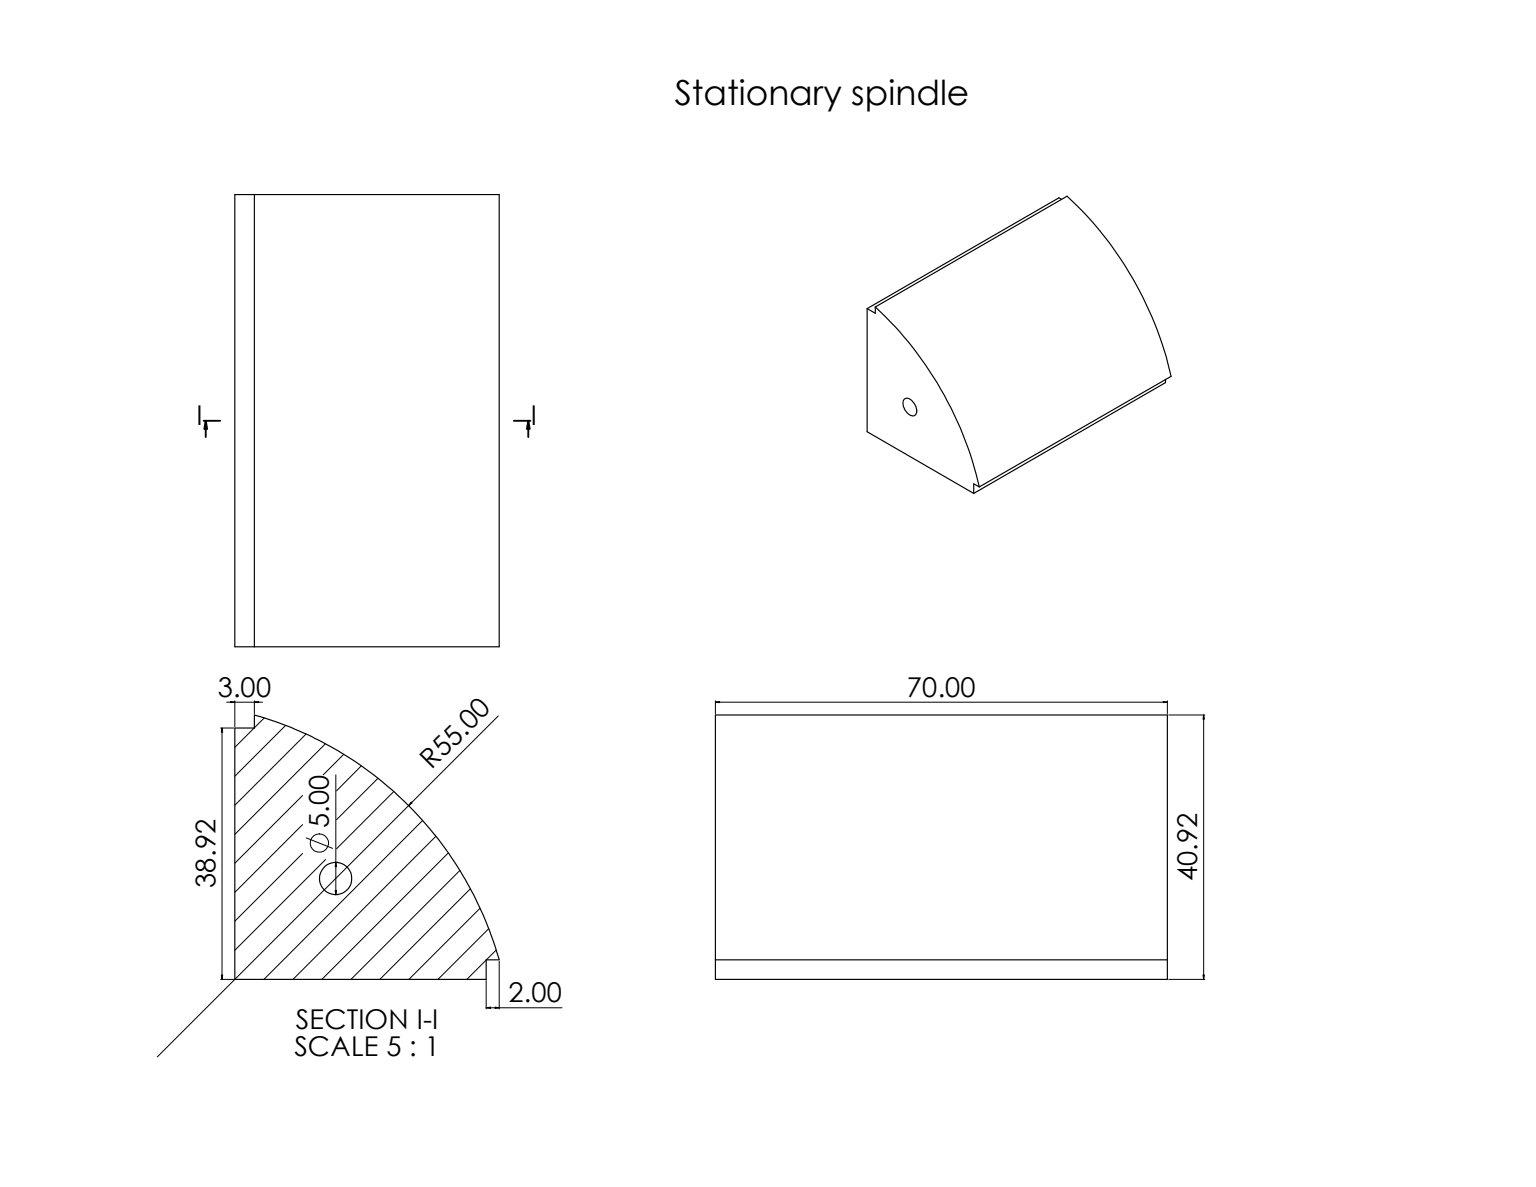
ISO-10303-21;
HEADER;
FILE_DESCRIPTION (('STEP AP214'),
    '1' );
FILE_NAME ('Stationary spindle.step',
    '2026-10-25T19:19:31',
    ( '' ),
    ( '' ),
    'SwSTEP 2.0',
    'SolidWorks 2025',
    '' );
FILE_SCHEMA (( 'AUTOMOTIVE_DESIGN' ));
ENDSEC;

DATA;
#4=DIRECTION ( 'NONE',  ( 1.000000000000000000, 1.776356839400250465E-15, 0.000000000000000000 ) ) ;
#22=CARTESIAN_POINT ( 'NONE',  ( 0.000000000000000000, 0.000000000000000000, -35.00000000000000000 ) ) ;
#73=AXIS2_PLACEMENT_3D ( 'NONE', #3304, #3763, #5645 ) ;
#75=MECHANICAL_DESIGN_GEOMETRIC_PRESENTATION_REPRESENTATION('',(#2849),#6131);
#80=DIRECTION ( 'NONE',  ( -0.000000000000000000, -0.000000000000000000, -1.000000000000000000 ) ) ;
#108=CARTESIAN_POINT ( 'NONE',  ( 12.00000000000000000, 12.00000000000000355, 35.00000000000000000 ) ) ;
#149=VERTEX_POINT ( 'NONE', #4105 ) ;
#164=EDGE_CURVE ( 'NONE', #4020, #3411, #5117, .T. ) ;
#178=SHAPE_DEFINITION_REPRESENTATION ( #473, #4081 ) ;
#253=EDGE_CURVE ( 'NONE', #2411, #1649, #3151, .T. ) ;
#263=ORIENTED_EDGE ( 'NONE', *, *, #5260, .F. ) ;
#271=ORIENTED_EDGE ( 'NONE', *, *, #5533, .F. ) ;
#308=DIRECTION ( 'NONE',  ( 1.000000000000000000, 0.000000000000000000, 0.000000000000000000 ) ) ;
#320=EDGE_CURVE ( 'NONE', #1017, #4020, #950, .T. ) ;
#327=DIRECTION ( 'NONE',  ( 0.000000000000000000, 0.000000000000000000, 1.000000000000000000 ) ) ;
#328=VERTEX_POINT ( 'NONE', #555 ) ;
#343=ORIENTED_EDGE ( 'NONE', *, *, #4753, .T. ) ;
#349=EDGE_LOOP ( 'NONE', ( #4550, #1268, #2494, #2612 ) ) ;
#376=CYLINDRICAL_SURFACE ( 'NONE', #2340, 2.499999999999998668 ) ;
#377=AXIS2_PLACEMENT_3D ( 'NONE', #1815, #1301, #327 ) ;
#383=FACE_OUTER_BOUND ( 'NONE', #5206, .T. ) ;
#397=( NAMED_UNIT ( * ) PLANE_ANGLE_UNIT ( ) SI_UNIT ( $, .RADIAN. ) );
#400=AXIS2_PLACEMENT_3D ( 'NONE', #1642, #1196, #3511 ) ;
#414=DIRECTION ( 'NONE',  ( 8.673617379883998001E-16, 1.000000000000000000, 0.000000000000000000 ) ) ;
#466=VECTOR ( 'NONE', #2853, 1000.000000000000000 ) ;
#468=ADVANCED_FACE ( 'NONE', ( #2082, #5872 ), #4008, .T. ) ;
#473=PRODUCT_DEFINITION_SHAPE ( 'NONE', 'NONE',  #5093 ) ;
#476=ADVANCED_FACE ( 'NONE', ( #3547 ), #1167, .F. ) ;
#509=CARTESIAN_POINT ( 'NONE',  ( 50.91502622129181788, 0.000000000000000000, 35.00000000000000000 ) ) ;
#520=ORIENTED_EDGE ( 'NONE', *, *, #3591, .F. ) ;
#527=CARTESIAN_POINT ( 'NONE',  ( 15.00000000000000000, 50.91502622129181788, -35.00000000000000000 ) ) ;
#544=CARTESIAN_POINT ( 'NONE',  ( 30.10043906316099083, 27.60043906316109386, -35.00000000000000000 ) ) ;
#550=( NAMED_UNIT ( * ) PLANE_ANGLE_UNIT ( ) SI_UNIT ( $, .RADIAN. ) );
#551=EDGE_LOOP ( 'NONE', ( #5803, #2026, #2863, #2751, #5984, #4013, #6009 ) ) ;
#555=CARTESIAN_POINT ( 'NONE',  ( 25.10043906316099083, 27.60043906316109386, 35.00000000000000000 ) ) ;
#568=CARTESIAN_POINT ( 'NONE',  ( -0.000000000000000000, 50.91502622129181788, -35.00000000000000000 ) ) ;
#650=ORIENTED_EDGE ( 'NONE', *, *, #4683, .F. ) ;
#667=ADVANCED_FACE ( 'NONE', ( #3633 ), #5550, .T. ) ;
#688=VERTEX_POINT ( 'NONE', #2707 ) ;
#706=CARTESIAN_POINT ( 'NONE',  ( 0.000000000000000000, 12.00000000000000355, 35.00000000000000000 ) ) ;
#720=VERTEX_POINT ( 'NONE', #3203 ) ;
#726=EDGE_LOOP ( 'NONE', ( #3570, #4220, #4699, #3819 ) ) ;
#751=EDGE_LOOP ( 'NONE', ( #4191, #5188, #5078, #271 ) ) ;
#755=CARTESIAN_POINT ( 'NONE',  ( 25.10043906316099083, 27.60043906316109386, -35.00000000000000000 ) ) ;
#781=DIRECTION ( 'NONE',  ( -0.000000000000000000, 0.000000000000000000, 1.000000000000000000 ) ) ;
#809=DIRECTION ( 'NONE',  ( -0.000000000000000000, -0.000000000000000000, -1.000000000000000000 ) ) ;
#829=PLANE ( 'NONE',  #4757 ) ;
#874=FACE_OUTER_BOUND ( 'NONE', #751, .T. ) ;
#896=CARTESIAN_POINT ( 'NONE',  ( 50.91502622129181788, 15.00000000000000355, 35.00000000000000000 ) ) ;
#922=DIRECTION ( 'NONE',  ( -1.000000000000000000, -8.673617379884027583E-15, 0.000000000000000000 ) ) ;
#923=( LENGTH_UNIT ( ) NAMED_UNIT ( * ) SI_UNIT ( .MILLI., .METRE. ) );
#950=LINE ( 'NONE', #2871, #1656 ) ;
#986=DIRECTION ( 'NONE',  ( 0.000000000000000000, 1.000000000000000000, -0.000000000000000000 ) ) ;
#995=AXIS2_PLACEMENT_3D ( 'NONE', #2420, #5267, #4 ) ;
#999=FACE_OUTER_BOUND ( 'NONE', #4574, .T. ) ;
#1017=VERTEX_POINT ( 'NONE', #4611 ) ;
#1024=LINE ( 'NONE', #5212, #2674 ) ;
#1036=EDGE_LOOP ( 'NONE', ( #3545, #2131, #2003, #343 ) ) ;
#1042=VERTEX_POINT ( 'NONE', #3696 ) ;
#1089=EDGE_CURVE ( 'NONE', #328, #5376, #1799, .T. ) ;
#1123=EDGE_CURVE ( 'NONE', #4796, #1042, #2187, .T. ) ;
#1143=ORIENTED_EDGE ( 'NONE', *, *, #1123, .T. ) ;
#1152=VECTOR ( 'NONE', #80, 1000.000000000000000 ) ;
#1167=CYLINDRICAL_SURFACE ( 'NONE', #400, 2.499999999999998668 ) ;
#1196=DIRECTION ( 'NONE',  ( -0.000000000000000000, -0.000000000000000000, -1.000000000000000000 ) ) ;
#1206=ORIENTED_EDGE ( 'NONE', *, *, #4650, .F. ) ;
#1222=EDGE_CURVE ( 'NONE', #3173, #149, #5703, .T. ) ;
#1229=LINE ( 'NONE', #4014, #5612 ) ;
#1243=ORIENTED_EDGE ( 'NONE', *, *, #5448, .T. ) ;
#1248=CARTESIAN_POINT ( 'NONE',  ( 52.91502622129182498, 15.00000000000001954, -35.00000000000000000 ) ) ;
#1262=ORIENTED_EDGE ( 'NONE', *, *, #5100, .T. ) ;
#1263=AXIS2_PLACEMENT_3D ( 'NONE', #509, #3316, #4204 ) ;
#1268=ORIENTED_EDGE ( 'NONE', *, *, #253, .T. ) ;
#1272=FACE_BOUND ( 'NONE', #4669, .T. ) ;
#1275=CARTESIAN_POINT ( 'NONE',  ( 0.000000000000000000, 50.91502622129181788, 35.00000000000000000 ) ) ;
#1278=PLANE ( 'NONE',  #1480 ) ;
#1295=ADVANCED_FACE ( 'NONE', ( #1993 ), #4736, .T. ) ;
#1301=DIRECTION ( 'NONE',  ( -1.000000000000000000, 0.000000000000000000, 0.000000000000000000 ) ) ;
#1345=VERTEX_POINT ( 'NONE', #5925 ) ;
#1354=CLOSED_SHELL ( 'NONE', ( #476, #1295, #3315, #667, #2484, #4606, #2119, #4414, #4024, #468, #2528 ) ) ;
#1413=EDGE_LOOP ( 'NONE', ( #5205, #2301, #5017, #1262 ) ) ;
#1452=VECTOR ( 'NONE', #414, 1000.000000000000000 ) ;
#1459=ORIENTED_EDGE ( 'NONE', *, *, #5260, .T. ) ;
#1480=AXIS2_PLACEMENT_3D ( 'NONE', #4135, #3179, #5087 ) ;
#1485=EDGE_CURVE ( 'NONE', #149, #5582, #5139, .T. ) ;
#1642=CARTESIAN_POINT ( 'NONE',  ( 27.60043906316099083, 27.60043906316109386, 35.00000000000000000 ) ) ;
#1649=VERTEX_POINT ( 'NONE', #544 ) ;
#1656=VECTOR ( 'NONE', #4326, 1000.000000000000000 ) ;
#1686=CARTESIAN_POINT ( 'NONE',  ( 15.00000000000000000, 50.91502622129181788, 35.00000000000000000 ) ) ;
#1706=LINE ( 'NONE', #5609, #2127 ) ;
#1747=( GEOMETRIC_REPRESENTATION_CONTEXT ( 3 ) GLOBAL_UNCERTAINTY_ASSIGNED_CONTEXT ( ( #1880 ) ) GLOBAL_UNIT_ASSIGNED_CONTEXT ( ( #923, #397, #5586 ) ) REPRESENTATION_CONTEXT ( 'NONE', 'WORKASPACE' ) );
#1781=ORIENTED_EDGE ( 'NONE', *, *, #2108, .T. ) ;
#1799=LINE ( 'NONE', #2212, #4144 ) ;
#1800=LINE ( 'NONE', #896, #1152 ) ;
#1815=CARTESIAN_POINT ( 'NONE',  ( 12.00000000000000000, 0.000000000000000000, 35.00000000000000000 ) ) ;
#1844=CARTESIAN_POINT ( 'NONE',  ( 50.91502622129181788, 0.000000000000000000, -35.00000000000000000 ) ) ;
#1847=EDGE_CURVE ( 'NONE', #720, #3173, #3504, .T. ) ;
#1862=VECTOR ( 'NONE', #5992, 1000.000000000000000 ) ;
#1871=AXIS2_PLACEMENT_3D ( 'NONE', #22, #4840, #2930 ) ;
#1880=UNCERTAINTY_MEASURE_WITH_UNIT (LENGTH_MEASURE( 1.000000000000000082E-05 ), #923, 'distance_accuracy_value', 'NONE');
#1908=CARTESIAN_POINT ( 'NONE',  ( 12.00000000000000000, 0.000000000000000000, -35.00000000000000000 ) ) ;
#1944=CARTESIAN_POINT ( 'NONE',  ( 12.00000000000000000, 50.91502622129181788, -35.00000000000000000 ) ) ;
#1946=PRODUCT_DEFINITION_CONTEXT ( 'detailed design', #2778, 'design' ) ;
#1993=FACE_OUTER_BOUND ( 'NONE', #5463, .T. ) ;
#2003=ORIENTED_EDGE ( 'NONE', *, *, #5024, .T. ) ;
#2026=ORIENTED_EDGE ( 'NONE', *, *, #1123, .F. ) ;
#2082=FACE_BOUND ( 'NONE', #2328, .T. ) ;
#2108=EDGE_CURVE ( 'NONE', #1042, #4214, #5689, .T. ) ;
#2119=ADVANCED_FACE ( 'NONE', ( #4686 ), #4342, .T. ) ;
#2126=EDGE_CURVE ( 'NONE', #3411, #4200, #3871, .T. ) ;
#2127=VECTOR ( 'NONE', #2742, 1000.000000000000000 ) ;
#2131=ORIENTED_EDGE ( 'NONE', *, *, #5100, .F. ) ;
#2133=AXIS2_PLACEMENT_3D ( 'NONE', #3258, #4207, #3289 ) ;
#2139=CIRCLE ( 'NONE', #2944, 2.499999999999998668 ) ;
#2153=MANIFOLD_SOLID_BREP ( 'Boss-Extrude5', #1354 ) ;
#2187=LINE ( 'NONE', #4076, #1862 ) ;
#2212=CARTESIAN_POINT ( 'NONE',  ( 25.10043906316099083, 27.60043906316109386, 35.00000000000000000 ) ) ;
#2259=VECTOR ( 'NONE', #5084, 1000.000000000000000 ) ;
#2263=VECTOR ( 'NONE', #5671, 1000.000000000000000 ) ;
#2276=SHAPE_REPRESENTATION_RELATIONSHIP ( 'NONE' , 'NONE' ,  #4081, #3579 ) ;
#2291=CARTESIAN_POINT ( 'NONE',  ( 30.10043906316099083, 27.60043906316109386, 35.00000000000000000 ) ) ;
#2301=ORIENTED_EDGE ( 'NONE', *, *, #320, .F. ) ;
#2316=DIRECTION ( 'NONE',  ( 0.000000000000000000, -1.000000000000000000, 0.000000000000000000 ) ) ;
#2328=EDGE_LOOP ( 'NONE', ( #1206, #650 ) ) ;
#2330=DIRECTION ( 'NONE',  ( 1.000000000000000000, 0.000000000000000000, 0.000000000000000000 ) ) ;
#2331=VECTOR ( 'NONE', #4361, 1000.000000000000000 ) ;
#2336=LINE ( 'NONE', #2470, #2331 ) ;
#2340=AXIS2_PLACEMENT_3D ( 'NONE', #5539, #2755, #3617 ) ;
#2387=DIRECTION ( 'NONE',  ( 0.000000000000000000, -0.000000000000000000, -1.000000000000000000 ) ) ;
#2397=EDGE_CURVE ( 'NONE', #5277, #4214, #3713, .T. ) ;
#2411=VERTEX_POINT ( 'NONE', #2291 ) ;
#2416=PLANE ( 'NONE',  #2723 ) ;
#2420=CARTESIAN_POINT ( 'NONE',  ( 0.000000000000000000, 0.000000000000000000, 35.00000000000000000 ) ) ;
#2470=CARTESIAN_POINT ( 'NONE',  ( 0.000000000000000000, 12.00000000000000355, -35.00000000000000000 ) ) ;
#2484=ADVANCED_FACE ( 'NONE', ( #5600 ), #5630, .T. ) ;
#2494=ORIENTED_EDGE ( 'NONE', *, *, #2773, .F. ) ;
#2514=DIRECTION ( 'NONE',  ( 1.000000000000000000, 0.000000000000000000, 0.000000000000000000 ) ) ;
#2528=ADVANCED_FACE ( 'NONE', ( #1272, #383 ), #829, .F. ) ;
#2553=CIRCLE ( 'NONE', #4959, 2.499999999999998668 ) ;
#2567=EDGE_CURVE ( 'NONE', #1042, #1017, #2577, .T. ) ;
#2577=CIRCLE ( 'NONE', #995, 55.00000000000002132 ) ;
#2599=EDGE_LOOP ( 'NONE', ( #4253, #2986, #1143, #1781 ) ) ;
#2612=ORIENTED_EDGE ( 'NONE', *, *, #1089, .F. ) ;
#2620=DIRECTION ( 'NONE',  ( -0.000000000000000000, 0.000000000000000000, 1.000000000000000000 ) ) ;
#2633=ORIENTED_EDGE ( 'NONE', *, *, #1485, .T. ) ;
#2674=VECTOR ( 'NONE', #5648, 1000.000000000000000 ) ;
#2704=DIRECTION ( 'NONE',  ( 1.000000000000000000, 0.000000000000000000, 0.000000000000000000 ) ) ;
#2707=CARTESIAN_POINT ( 'NONE',  ( 50.91502622129181788, 15.00000000000000355, 35.00000000000000000 ) ) ;
#2723=AXIS2_PLACEMENT_3D ( 'NONE', #4305, #5289, #2387 ) ;
#2735=FACE_OUTER_BOUND ( 'NONE', #1413, .T. ) ;
#2738=VECTOR ( 'NONE', #4018, 1000.000000000000000 ) ;
#2742=DIRECTION ( 'NONE',  ( 0.000000000000000000, -1.000000000000000000, 0.000000000000000000 ) ) ;
#2751=ORIENTED_EDGE ( 'NONE', *, *, #1222, .F. ) ;
#2755=DIRECTION ( 'NONE',  ( -0.000000000000000000, -0.000000000000000000, -1.000000000000000000 ) ) ;
#2773=EDGE_CURVE ( 'NONE', #5376, #1649, #2553, .T. ) ;
#2778=APPLICATION_CONTEXT ( 'automotive_design' ) ;
#2783=ORIENTED_EDGE ( 'NONE', *, *, #2397, .T. ) ;
#2816=CARTESIAN_POINT ( 'NONE',  ( 15.00000000000000178, 52.91502622129183209, 35.00000000000000000 ) ) ;
#2845=PRODUCT ( 'Stationary spindle', 'Stationary spindle', '', ( #3575 ) ) ;
#2849=STYLED_ITEM('',(#6170),#2153);
#2853=DIRECTION ( 'NONE',  ( 0.000000000000000000, 1.000000000000000000, -0.000000000000000000 ) ) ;
#2863=ORIENTED_EDGE ( 'NONE', *, *, #4845, .F. ) ;
#2871=CARTESIAN_POINT ( 'NONE',  ( 52.91502622129182498, 15.00000000000001954, 35.00000000000000000 ) ) ;
#2896=ORIENTED_EDGE ( 'NONE', *, *, #5448, .F. ) ;
#2910=CARTESIAN_POINT ( 'NONE',  ( 27.60043906316099083, 27.60043906316109386, 35.00000000000000000 ) ) ;
#2930=DIRECTION ( 'NONE',  ( 1.000000000000000000, 1.776356839400250465E-15, 0.000000000000000000 ) ) ;
#2944=AXIS2_PLACEMENT_3D ( 'NONE', #5384, #781, #3932 ) ;
#2986=ORIENTED_EDGE ( 'NONE', *, *, #5982, .F. ) ;
#3053=DIRECTION ( 'NONE',  ( 1.000000000000000000, 0.000000000000000000, 0.000000000000000000 ) ) ;
#3056=VECTOR ( 'NONE', #922, 1000.000000000000000 ) ;
#3151=LINE ( 'NONE', #5778, #4153 ) ;
#3168=ORIENTED_EDGE ( 'NONE', *, *, #2108, .F. ) ;
#3173=VERTEX_POINT ( 'NONE', #4459 ) ;
#3174=DIRECTION ( 'NONE',  ( -0.000000000000000000, 0.000000000000000000, 1.000000000000000000 ) ) ;
#3179=DIRECTION ( 'NONE',  ( -1.000000000000000000, 8.673617379883998001E-16, 0.000000000000000000 ) ) ;
#3203=CARTESIAN_POINT ( 'NONE',  ( 50.91502622129181788, 12.00000000000000355, 35.00000000000000000 ) ) ;
#3228=CARTESIAN_POINT ( 'NONE',  ( 0.000000000000000000, 0.000000000000000000, -35.00000000000000000 ) ) ;
#3258=CARTESIAN_POINT ( 'NONE',  ( 27.60043906316099083, 27.60043906316109386, -35.00000000000000000 ) ) ;
#3260=AXIS2_PLACEMENT_3D ( 'NONE', #5642, #3274, #5179 ) ;
#3263=CARTESIAN_POINT ( 'NONE',  ( 14.99999999999995559, -1.301042606982595854E-14, -35.00000000000000000 ) ) ;
#3274=DIRECTION ( 'NONE',  ( -0.000000000000000000, -0.000000000000000000, -1.000000000000000000 ) ) ;
#3289=DIRECTION ( 'NONE',  ( 1.000000000000000000, 0.000000000000000000, 0.000000000000000000 ) ) ;
#3302=CARTESIAN_POINT ( 'NONE',  ( 12.00000000000000000, 0.000000000000000000, 35.00000000000000000 ) ) ;
#3304=CARTESIAN_POINT ( 'NONE',  ( 0.000000000000000000, 0.000000000000000000, 0.000000000000000000 ) ) ;
#3315=ADVANCED_FACE ( 'NONE', ( #5497 ), #1278, .T. ) ;
#3316=DIRECTION ( 'NONE',  ( 1.000000000000000000, 0.000000000000000000, -0.000000000000000000 ) ) ;
#3320=ORIENTED_EDGE ( 'NONE', *, *, #4753, .F. ) ;
#3350=EDGE_CURVE ( 'NONE', #3173, #1345, #4731, .T. ) ;
#3402=CARTESIAN_POINT ( 'NONE',  ( 15.00000000000000000, 50.91502622129181788, 35.00000000000000000 ) ) ;
#3411=VERTEX_POINT ( 'NONE', #5638 ) ;
#3504=LINE ( 'NONE', #706, #3723 ) ;
#3511=DIRECTION ( 'NONE',  ( -1.000000000000000000, 0.000000000000000000, 0.000000000000000000 ) ) ;
#3516=CIRCLE ( 'NONE', #5025, 2.499999999999998668 ) ;
#3532=VECTOR ( 'NONE', #5287, 1000.000000000000000 ) ;
#3536=PRODUCT_DEFINITION_FORMATION_WITH_SPECIFIED_SOURCE ( 'ANY', '', #2845, .NOT_KNOWN. ) ;
#3545=ORIENTED_EDGE ( 'NONE', *, *, #2126, .F. ) ;
#3547=FACE_OUTER_BOUND ( 'NONE', #349, .T. ) ;
#3570=ORIENTED_EDGE ( 'NONE', *, *, #4538, .F. ) ;
#3573=CARTESIAN_POINT ( 'NONE',  ( 12.00000000000000000, 50.91502622129181788, 35.00000000000000000 ) ) ;
#3575=PRODUCT_CONTEXT ( 'NONE', #5891, 'mechanical' ) ;
#3579=ADVANCED_BREP_SHAPE_REPRESENTATION ( '', ( #2153, #73 ), #1747 ) ;
#3591=EDGE_CURVE ( 'NONE', #4214, #4020, #5569, .T. ) ;
#3617=DIRECTION ( 'NONE',  ( -1.000000000000000000, 0.000000000000000000, 0.000000000000000000 ) ) ;
#3633=FACE_OUTER_BOUND ( 'NONE', #726, .T. ) ;
#3653=EDGE_CURVE ( 'NONE', #1017, #688, #1024, .T. ) ;
#3696=CARTESIAN_POINT ( 'NONE',  ( 15.00000000000000178, 52.91502622129183209, 35.00000000000000000 ) ) ;
#3713=LINE ( 'NONE', #3263, #1452 ) ;
#3722=CARTESIAN_POINT ( 'NONE',  ( 27.60043906316099083, 27.60043906316109386, -35.00000000000000000 ) ) ;
#3723=VECTOR ( 'NONE', #4476, 1000.000000000000000 ) ;
#3739=AXIS2_PLACEMENT_3D ( 'NONE', #3918, #2620, #3053 ) ;
#3763=DIRECTION ( 'NONE',  ( 0.000000000000000000, 0.000000000000000000, 1.000000000000000000 ) ) ;
#3771=ORIENTED_EDGE ( 'NONE', *, *, #4538, .T. ) ;
#3817=CIRCLE ( 'NONE', #2133, 2.499999999999998668 ) ;
#3819=ORIENTED_EDGE ( 'NONE', *, *, #5982, .T. ) ;
#3845=EDGE_LOOP ( 'NONE', ( #2896, #5965, #5999, #2633 ) ) ;
#3871=LINE ( 'NONE', #1844, #4743 ) ;
#3889=DIRECTION ( 'NONE',  ( -0.000000000000000000, -0.000000000000000000, -1.000000000000000000 ) ) ;
#3918=CARTESIAN_POINT ( 'NONE',  ( 0.000000000000000000, 0.000000000000000000, 35.00000000000000000 ) ) ;
#3932=DIRECTION ( 'NONE',  ( 1.000000000000000000, 0.000000000000000000, 0.000000000000000000 ) ) ;
#4008=PLANE ( 'NONE',  #3739 ) ;
#4013=ORIENTED_EDGE ( 'NONE', *, *, #5024, .F. ) ;
#4014=CARTESIAN_POINT ( 'NONE',  ( 0.000000000000000000, 50.91502622129181788, 35.00000000000000000 ) ) ;
#4018=DIRECTION ( 'NONE',  ( -0.000000000000000000, -0.000000000000000000, -1.000000000000000000 ) ) ;
#4020=VERTEX_POINT ( 'NONE', #1248 ) ;
#4024=ADVANCED_FACE ( 'NONE', ( #2735 ), #5143, .T. ) ;
#4030=ORIENTED_EDGE ( 'NONE', *, *, #2773, .T. ) ;
#4076=CARTESIAN_POINT ( 'NONE',  ( 14.99999999999995559, -1.301042606982595854E-14, 35.00000000000000000 ) ) ;
#4081=SHAPE_REPRESENTATION ( 'Stationary spindle', ( #73 ), #1747 ) ;
#4105=CARTESIAN_POINT ( 'NONE',  ( 12.00000000000000000, 50.91502622129181788, 35.00000000000000000 ) ) ;
#4135=CARTESIAN_POINT ( 'NONE',  ( 14.99999999999995559, -1.301042606982595854E-14, 35.00000000000000000 ) ) ;
#4144=VECTOR ( 'NONE', #809, 1000.000000000000000 ) ;
#4153=VECTOR ( 'NONE', #3889, 1000.000000000000000 ) ;
#4191=ORIENTED_EDGE ( 'NONE', *, *, #253, .F. ) ;
#4200=VERTEX_POINT ( 'NONE', #5365 ) ;
#4202=ORIENTED_EDGE ( 'NONE', *, *, #1847, .T. ) ;
#4204=DIRECTION ( 'NONE',  ( -0.000000000000000000, 0.000000000000000000, -1.000000000000000000 ) ) ;
#4207=DIRECTION ( 'NONE',  ( -0.000000000000000000, 0.000000000000000000, 1.000000000000000000 ) ) ;
#4214=VERTEX_POINT ( 'NONE', #5797 ) ;
#4220=ORIENTED_EDGE ( 'NONE', *, *, #1485, .F. ) ;
#4231=VECTOR ( 'NONE', #4786, 1000.000000000000000 ) ;
#4253=ORIENTED_EDGE ( 'NONE', *, *, #2397, .F. ) ;
#4305=CARTESIAN_POINT ( 'NONE',  ( 0.000000000000000000, 12.00000000000000355, 35.00000000000000000 ) ) ;
#4326=DIRECTION ( 'NONE',  ( -0.000000000000000000, -0.000000000000000000, -1.000000000000000000 ) ) ;
#4342=PLANE ( 'NONE',  #1263 ) ;
#4361=DIRECTION ( 'NONE',  ( -1.000000000000000000, 0.000000000000000000, 0.000000000000000000 ) ) ;
#4374=LINE ( 'NONE', #568, #5432 ) ;
#4414=ADVANCED_FACE ( 'NONE', ( #874 ), #376, .F. ) ;
#4459=CARTESIAN_POINT ( 'NONE',  ( 12.00000000000000000, 12.00000000000000355, 35.00000000000000000 ) ) ;
#4476=DIRECTION ( 'NONE',  ( -1.000000000000000000, 0.000000000000000000, 0.000000000000000000 ) ) ;
#4538=EDGE_CURVE ( 'NONE', #5582, #5277, #4374, .T. ) ;
#4540=ORIENTED_EDGE ( 'NONE', *, *, #164, .T. ) ;
#4550=ORIENTED_EDGE ( 'NONE', *, *, #4650, .T. ) ;
#4574=EDGE_LOOP ( 'NONE', ( #263, #3320, #4202, #5299 ) ) ;
#4604=DIRECTION ( 'NONE',  ( 0.000000000000000000, 1.000000000000000000, 0.000000000000000000 ) ) ;
#4606=ADVANCED_FACE ( 'NONE', ( #999 ), #2416, .T. ) ;
#4611=CARTESIAN_POINT ( 'NONE',  ( 52.91502622129182498, 15.00000000000001954, 35.00000000000000000 ) ) ;
#4638=DIRECTION ( 'NONE',  ( 1.000000000000000000, 8.673617379884027583E-15, 0.000000000000000000 ) ) ;
#4647=AXIS2_PLACEMENT_3D ( 'NONE', #1275, #4604, #5141 ) ;
#4650=EDGE_CURVE ( 'NONE', #328, #2411, #3516, .T. ) ;
#4669=EDGE_LOOP ( 'NONE', ( #4030, #4888 ) ) ;
#4683=EDGE_CURVE ( 'NONE', #2411, #328, #2139, .T. ) ;
#4686=FACE_OUTER_BOUND ( 'NONE', #1036, .T. ) ;
#4688=UNCERTAINTY_MEASURE_WITH_UNIT (LENGTH_MEASURE( 1.000000000000000082E-05 ), #5652, 'distance_accuracy_value', 'NONE');
#4699=ORIENTED_EDGE ( 'NONE', *, *, #4845, .T. ) ;
#4731=LINE ( 'NONE', #108, #2263 ) ;
#4736=CYLINDRICAL_SURFACE ( 'NONE', #3260, 55.00000000000002132 ) ;
#4743=VECTOR ( 'NONE', #2316, 1000.000000000000000 ) ;
#4753=EDGE_CURVE ( 'NONE', #720, #4200, #5410, .T. ) ;
#4757=AXIS2_PLACEMENT_3D ( 'NONE', #3228, #3174, #2704 ) ;
#4786=DIRECTION ( 'NONE',  ( -0.000000000000000000, -0.000000000000000000, -1.000000000000000000 ) ) ;
#4796=VERTEX_POINT ( 'NONE', #1686 ) ;
#4840=DIRECTION ( 'NONE',  ( 0.000000000000000000, -0.000000000000000000, -1.000000000000000000 ) ) ;
#4845=EDGE_CURVE ( 'NONE', #149, #4796, #1229, .T. ) ;
#4888=ORIENTED_EDGE ( 'NONE', *, *, #5533, .T. ) ;
#4959=AXIS2_PLACEMENT_3D ( 'NONE', #3722, #6105, #2330 ) ;
#5017=ORIENTED_EDGE ( 'NONE', *, *, #3653, .T. ) ;
#5024=EDGE_CURVE ( 'NONE', #688, #720, #1706, .T. ) ;
#5025=AXIS2_PLACEMENT_3D ( 'NONE', #2910, #5787, #5882 ) ;
#5032=AXIS2_PLACEMENT_3D ( 'NONE', #5496, #5110, #4638 ) ;
#5048=ORIENTED_EDGE ( 'NONE', *, *, #2126, .T. ) ;
#5058=ORIENTED_EDGE ( 'NONE', *, *, #2567, .T. ) ;
#5078=ORIENTED_EDGE ( 'NONE', *, *, #1089, .T. ) ;
#5084=DIRECTION ( 'NONE',  ( -0.000000000000000000, -0.000000000000000000, -1.000000000000000000 ) ) ;
#5087=DIRECTION ( 'NONE',  ( -8.673617379883998001E-16, -1.000000000000000000, 0.000000000000000000 ) ) ;
#5093=PRODUCT_DEFINITION ( 'UNKNOWN', '', #3536, #1946 ) ;
#5100=EDGE_CURVE ( 'NONE', #688, #3411, #1800, .T. ) ;
#5110=DIRECTION ( 'NONE',  ( 8.673617379884027583E-15, -1.000000000000000000, 0.000000000000000000 ) ) ;
#5117=LINE ( 'NONE', #6081, #3056 ) ;
#5139=LINE ( 'NONE', #3573, #2259 ) ;
#5141=DIRECTION ( 'NONE',  ( 0.000000000000000000, -0.000000000000000000, 1.000000000000000000 ) ) ;
#5143=PLANE ( 'NONE',  #5032 ) ;
#5179=DIRECTION ( 'NONE',  ( -1.000000000000000000, 0.000000000000000000, 0.000000000000000000 ) ) ;
#5188=ORIENTED_EDGE ( 'NONE', *, *, #4683, .T. ) ;
#5205=ORIENTED_EDGE ( 'NONE', *, *, #164, .F. ) ;
#5206=EDGE_LOOP ( 'NONE', ( #5543, #4540, #5048, #1459, #1243, #3771, #2783 ) ) ;
#5212=CARTESIAN_POINT ( 'NONE',  ( -1.301042606982566193E-13, 14.99999999999956124, 35.00000000000000000 ) ) ;
#5260=EDGE_CURVE ( 'NONE', #4200, #1345, #2336, .T. ) ;
#5267=DIRECTION ( 'NONE',  ( 0.000000000000000000, -0.000000000000000000, -1.000000000000000000 ) ) ;
#5277=VERTEX_POINT ( 'NONE', #527 ) ;
#5287=DIRECTION ( 'NONE',  ( -0.000000000000000000, -0.000000000000000000, -1.000000000000000000 ) ) ;
#5289=DIRECTION ( 'NONE',  ( 0.000000000000000000, -1.000000000000000000, 0.000000000000000000 ) ) ;
#5299=ORIENTED_EDGE ( 'NONE', *, *, #3350, .T. ) ;
#5304=ORIENTED_EDGE ( 'NONE', *, *, #320, .T. ) ;
#5365=CARTESIAN_POINT ( 'NONE',  ( 50.91502622129181788, 12.00000000000000355, -35.00000000000000000 ) ) ;
#5376=VERTEX_POINT ( 'NONE', #755 ) ;
#5384=CARTESIAN_POINT ( 'NONE',  ( 27.60043906316099083, 27.60043906316109386, 35.00000000000000000 ) ) ;
#5410=LINE ( 'NONE', #5477, #2738 ) ;
#5432=VECTOR ( 'NONE', #2514, 1000.000000000000000 ) ;
#5448=EDGE_CURVE ( 'NONE', #1345, #5582, #6092, .T. ) ;
#5463=EDGE_LOOP ( 'NONE', ( #520, #3168, #5058, #5304 ) ) ;
#5477=CARTESIAN_POINT ( 'NONE',  ( 50.91502622129181788, 12.00000000000000355, 35.00000000000000000 ) ) ;
#5496=CARTESIAN_POINT ( 'NONE',  ( -1.301042606982566193E-13, 14.99999999999956124, 35.00000000000000000 ) ) ;
#5497=FACE_OUTER_BOUND ( 'NONE', #2599, .T. ) ;
#5533=EDGE_CURVE ( 'NONE', #1649, #5376, #3817, .T. ) ;
#5539=CARTESIAN_POINT ( 'NONE',  ( 27.60043906316099083, 27.60043906316109386, 35.00000000000000000 ) ) ;
#5543=ORIENTED_EDGE ( 'NONE', *, *, #3591, .T. ) ;
#5550=PLANE ( 'NONE',  #4647 ) ;
#5569=CIRCLE ( 'NONE', #1871, 55.00000000000002132 ) ;
#5582=VERTEX_POINT ( 'NONE', #1944 ) ;
#5586=( NAMED_UNIT ( * ) SI_UNIT ( $, .STERADIAN. ) SOLID_ANGLE_UNIT ( ) );
#5600=FACE_OUTER_BOUND ( 'NONE', #3845, .T. ) ;
#5609=CARTESIAN_POINT ( 'NONE',  ( 50.91502622129181788, 0.000000000000000000, 35.00000000000000000 ) ) ;
#5612=VECTOR ( 'NONE', #308, 1000.000000000000000 ) ;
#5630=PLANE ( 'NONE',  #377 ) ;
#5638=CARTESIAN_POINT ( 'NONE',  ( 50.91502622129181788, 15.00000000000000355, -35.00000000000000000 ) ) ;
#5642=CARTESIAN_POINT ( 'NONE',  ( 0.000000000000000000, 0.000000000000000000, 35.00000000000000000 ) ) ;
#5645=DIRECTION ( 'NONE',  ( 1.000000000000000000, 0.000000000000000000, 0.000000000000000000 ) ) ;
#5648=DIRECTION ( 'NONE',  ( -1.000000000000000000, -8.673617379884027583E-15, 0.000000000000000000 ) ) ;
#5652=( LENGTH_UNIT ( ) NAMED_UNIT ( * ) SI_UNIT ( .MILLI., .METRE. ) );
#5657=VECTOR ( 'NONE', #986, 1000.000000000000000 ) ;
#5671=DIRECTION ( 'NONE',  ( -0.000000000000000000, -0.000000000000000000, -1.000000000000000000 ) ) ;
#5689=LINE ( 'NONE', #2816, #4231 ) ;
#5703=LINE ( 'NONE', #3302, #5657 ) ;
#5750=LINE ( 'NONE', #3402, #3532 ) ;
#5778=CARTESIAN_POINT ( 'NONE',  ( 30.10043906316099083, 27.60043906316109386, 35.00000000000000000 ) ) ;
#5787=DIRECTION ( 'NONE',  ( -0.000000000000000000, 0.000000000000000000, 1.000000000000000000 ) ) ;
#5797=CARTESIAN_POINT ( 'NONE',  ( 15.00000000000000178, 52.91502622129183209, -35.00000000000000000 ) ) ;
#5803=ORIENTED_EDGE ( 'NONE', *, *, #2567, .F. ) ;
#5835=( NAMED_UNIT ( * ) SI_UNIT ( $, .STERADIAN. ) SOLID_ANGLE_UNIT ( ) );
#5872=FACE_OUTER_BOUND ( 'NONE', #551, .T. ) ;
#5882=DIRECTION ( 'NONE',  ( 1.000000000000000000, 0.000000000000000000, 0.000000000000000000 ) ) ;
#5891=APPLICATION_CONTEXT ( 'automotive_design' ) ;
#5925=CARTESIAN_POINT ( 'NONE',  ( 12.00000000000000000, 12.00000000000000355, -35.00000000000000000 ) ) ;
#5965=ORIENTED_EDGE ( 'NONE', *, *, #3350, .F. ) ;
#5982=EDGE_CURVE ( 'NONE', #4796, #5277, #5750, .T. ) ;
#5984=ORIENTED_EDGE ( 'NONE', *, *, #1847, .F. ) ;
#5992=DIRECTION ( 'NONE',  ( 8.673617379883998001E-16, 1.000000000000000000, 0.000000000000000000 ) ) ;
#5999=ORIENTED_EDGE ( 'NONE', *, *, #1222, .T. ) ;
#6009=ORIENTED_EDGE ( 'NONE', *, *, #3653, .F. ) ;
#6081=CARTESIAN_POINT ( 'NONE',  ( -1.301042606982566193E-13, 14.99999999999956124, -35.00000000000000000 ) ) ;
#6092=LINE ( 'NONE', #1908, #466 ) ;
#6105=DIRECTION ( 'NONE',  ( -0.000000000000000000, 0.000000000000000000, 1.000000000000000000 ) ) ;
#6131=( GEOMETRIC_REPRESENTATION_CONTEXT ( 3 ) GLOBAL_UNCERTAINTY_ASSIGNED_CONTEXT ( ( #4688 ) ) GLOBAL_UNIT_ASSIGNED_CONTEXT ( ( #5652, #550, #5835 ) ) REPRESENTATION_CONTEXT ( 'NONE', 'WORKASPACE' ) );
#6164=COLOUR_RGB('Light Blue',0.38,0.62,0.78);
#6165=FILL_AREA_STYLE_COLOUR('',#6164);
#6166=FILL_AREA_STYLE('',(#6165));
#6167=SURFACE_STYLE_FILL_AREA(#6166);
#6168=SURFACE_SIDE_STYLE('',(#6167));
#6169=SURFACE_STYLE_USAGE(.BOTH.,#6168);
#6170=PRESENTATION_STYLE_ASSIGNMENT((#6169));
ENDSEC;
END-ISO-10303-21;
